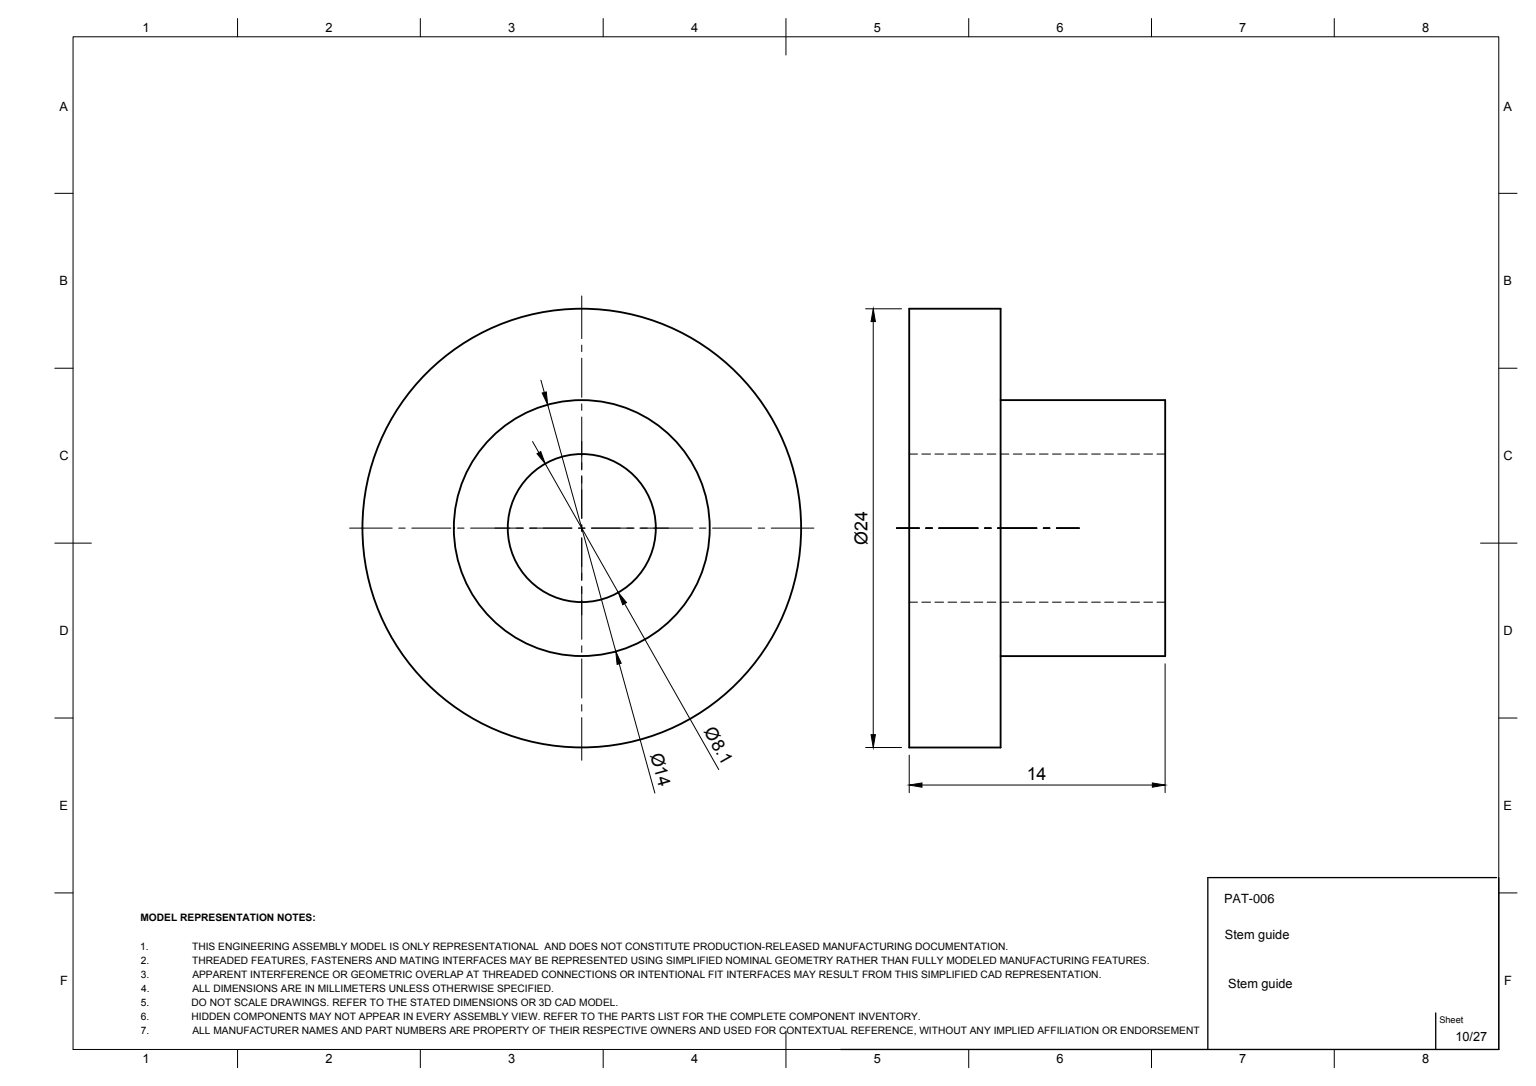
ISO-10303-21;
HEADER;
/* Generated by software containing ST-Developer
 * from STEP Tools, Inc. (www.steptools.com) 
 */

FILE_DESCRIPTION(
/* description */ ('Ball-type isolation valve (generic)'),
/* implementation_level */ '2;1');

FILE_NAME(
/* name */ 'Stem guide.step',
/* time_stamp */ '2026-10-27T10:53:05-07:00',
/* author */ (''),
/* organization */ (''),
/* preprocessor_version */ 'ST-DEVELOPER v20.2',
/* originating_system */ 'Autodesk Translation Framework v15.17.0.0',
/* authorisation */ '');

FILE_SCHEMA (('AUTOMOTIVE_DESIGN { 1 0 10303 214 3 1 1 }'));
ENDSEC;

DATA;
#10=MECHANICAL_DESIGN_GEOMETRIC_PRESENTATION_REPRESENTATION('',(#282),#7425);
#230=SHAPE_REPRESENTATION_RELATIONSHIP('SRR','None',#7540,#256);
#256=ADVANCED_BREP_SHAPE_REPRESENTATION('',(#308),#7403);
#282=STYLED_ITEM('',(#7737),#308);
#308=MANIFOLD_SOLID_BREP('Body1',#4087);
#373=FACE_BOUND('',#939,.T.);
#374=FACE_BOUND('',#942,.T.);
#375=FACE_BOUND('',#946,.T.);
#456=PLANE('',#4536);
#457=PLANE('',#4541);
#458=PLANE('',#4547);
#647=FACE_OUTER_BOUND('',#938,.T.);
#648=FACE_OUTER_BOUND('',#940,.T.);
#649=FACE_OUTER_BOUND('',#941,.T.);
#650=FACE_OUTER_BOUND('',#943,.T.);
#651=FACE_OUTER_BOUND('',#944,.T.);
#652=FACE_OUTER_BOUND('',#945,.T.);
#938=EDGE_LOOP('',(#3071));
#939=EDGE_LOOP('',(#3072));
#940=EDGE_LOOP('',(#3073,#3074,#3075,#3076));
#941=EDGE_LOOP('',(#3077));
#942=EDGE_LOOP('',(#3078));
#943=EDGE_LOOP('',(#3079,#3080,#3081,#3082));
#944=EDGE_LOOP('',(#3083,#3084,#3085,#3086));
#945=EDGE_LOOP('',(#3087));
#946=EDGE_LOOP('',(#3088));
#1251=LINE('',#6532,#1559);
#1252=LINE('',#6538,#1560);
#1253=LINE('',#6542,#1561);
#1559=VECTOR('',#5268,1.2);
#1560=VECTOR('',#5275,0.405);
#1561=VECTOR('',#5280,0.7);
#1843=CIRCLE('',#4537,1.2);
#1844=CIRCLE('',#4538,0.7);
#1845=CIRCLE('',#4540,1.2);
#1846=CIRCLE('',#4542,0.405);
#1847=CIRCLE('',#4544,0.405);
#1848=CIRCLE('',#4546,0.7);
#2056=VERTEX_POINT('',#6525);
#2057=VERTEX_POINT('',#6527);
#2058=VERTEX_POINT('',#6530);
#2059=VERTEX_POINT('',#6534);
#2060=VERTEX_POINT('',#6537);
#2061=VERTEX_POINT('',#6541);
#2428=EDGE_CURVE('',#2056,#2056,#1843,.T.);
#2429=EDGE_CURVE('',#2057,#2057,#1844,.T.);
#2430=EDGE_CURVE('',#2058,#2058,#1845,.T.);
#2431=EDGE_CURVE('',#2058,#2056,#1251,.T.);
#2432=EDGE_CURVE('',#2059,#2059,#1846,.T.);
#2433=EDGE_CURVE('',#2059,#2060,#1252,.T.);
#2434=EDGE_CURVE('',#2060,#2060,#1847,.T.);
#2435=EDGE_CURVE('',#2057,#2061,#1253,.T.);
#2436=EDGE_CURVE('',#2061,#2061,#1848,.T.);
#3071=ORIENTED_EDGE('',*,*,#2428,.F.);
#3072=ORIENTED_EDGE('',*,*,#2429,.T.);
#3073=ORIENTED_EDGE('',*,*,#2430,.F.);
#3074=ORIENTED_EDGE('',*,*,#2431,.T.);
#3075=ORIENTED_EDGE('',*,*,#2428,.T.);
#3076=ORIENTED_EDGE('',*,*,#2431,.F.);
#3077=ORIENTED_EDGE('',*,*,#2430,.T.);
#3078=ORIENTED_EDGE('',*,*,#2432,.T.);
#3079=ORIENTED_EDGE('',*,*,#2432,.F.);
#3080=ORIENTED_EDGE('',*,*,#2433,.T.);
#3081=ORIENTED_EDGE('',*,*,#2434,.T.);
#3082=ORIENTED_EDGE('',*,*,#2433,.F.);
#3083=ORIENTED_EDGE('',*,*,#2429,.F.);
#3084=ORIENTED_EDGE('',*,*,#2435,.T.);
#3085=ORIENTED_EDGE('',*,*,#2436,.T.);
#3086=ORIENTED_EDGE('',*,*,#2435,.F.);
#3087=ORIENTED_EDGE('',*,*,#2436,.F.);
#3088=ORIENTED_EDGE('',*,*,#2434,.F.);
#3792=CYLINDRICAL_SURFACE('',#4539,1.2);
#3793=CYLINDRICAL_SURFACE('',#4543,0.405);
#3794=CYLINDRICAL_SURFACE('',#4545,0.7);
#3901=ADVANCED_FACE('',(#647,#373),#456,.F.);
#3902=ADVANCED_FACE('',(#648),#3792,.T.);
#3903=ADVANCED_FACE('',(#649,#374),#457,.T.);
#3904=ADVANCED_FACE('',(#650),#3793,.F.);
#3905=ADVANCED_FACE('',(#651),#3794,.T.);
#3906=ADVANCED_FACE('',(#652,#375),#458,.F.);
#4087=CLOSED_SHELL('',(#3901,#3902,#3903,#3904,#3905,#3906));
#4535=AXIS2_PLACEMENT_3D('',#6523,#5256,#5257);
#4536=AXIS2_PLACEMENT_3D('',#6524,#5258,#5259);
#4537=AXIS2_PLACEMENT_3D('',#6526,#5260,#5261);
#4538=AXIS2_PLACEMENT_3D('',#6528,#5262,#5263);
#4539=AXIS2_PLACEMENT_3D('',#6529,#5264,#5265);
#4540=AXIS2_PLACEMENT_3D('',#6531,#5266,#5267);
#4541=AXIS2_PLACEMENT_3D('',#6533,#5269,#5270);
#4542=AXIS2_PLACEMENT_3D('',#6535,#5271,#5272);
#4543=AXIS2_PLACEMENT_3D('',#6536,#5273,#5274);
#4544=AXIS2_PLACEMENT_3D('',#6539,#5276,#5277);
#4545=AXIS2_PLACEMENT_3D('',#6540,#5278,#5279);
#4546=AXIS2_PLACEMENT_3D('',#6543,#5281,#5282);
#4547=AXIS2_PLACEMENT_3D('',#6544,#5283,#5284);
#5256=DIRECTION('axis',(0.,0.,1.));
#5257=DIRECTION('refdir',(1.,0.,0.));
#5258=DIRECTION('center_axis',(0.,0.,1.));
#5259=DIRECTION('ref_axis',(1.,0.,0.));
#5260=DIRECTION('center_axis',(0.,0.,1.));
#5261=DIRECTION('ref_axis',(1.,0.,0.));
#5262=DIRECTION('center_axis',(0.,0.,1.));
#5263=DIRECTION('ref_axis',(1.,0.,0.));
#5264=DIRECTION('center_axis',(0.,0.,1.));
#5265=DIRECTION('ref_axis',(1.,0.,0.));
#5266=DIRECTION('center_axis',(0.,0.,1.));
#5267=DIRECTION('ref_axis',(1.,0.,0.));
#5268=DIRECTION('',(0.,0.,-1.));
#5269=DIRECTION('center_axis',(0.,0.,1.));
#5270=DIRECTION('ref_axis',(1.,0.,0.));
#5271=DIRECTION('center_axis',(0.,0.,-1.));
#5272=DIRECTION('ref_axis',(1.,0.,0.));
#5273=DIRECTION('center_axis',(0.,0.,1.));
#5274=DIRECTION('ref_axis',(1.,0.,0.));
#5275=DIRECTION('',(0.,0.,-1.));
#5276=DIRECTION('center_axis',(0.,0.,-1.));
#5277=DIRECTION('ref_axis',(1.,0.,0.));
#5278=DIRECTION('center_axis',(0.,0.,1.));
#5279=DIRECTION('ref_axis',(1.,0.,0.));
#5280=DIRECTION('',(0.,0.,-1.));
#5281=DIRECTION('center_axis',(0.,0.,1.));
#5282=DIRECTION('ref_axis',(1.,0.,0.));
#5283=DIRECTION('center_axis',(0.,0.,1.));
#5284=DIRECTION('ref_axis',(1.,0.,0.));
#6523=CARTESIAN_POINT('',(0.,0.,0.));
#6524=CARTESIAN_POINT('Origin',(0.,0.,7.5));
#6525=CARTESIAN_POINT('',(-1.2,-1.46957615897682E-16,7.5));
#6526=CARTESIAN_POINT('Origin',(0.,0.,7.5));
#6527=CARTESIAN_POINT('',(-0.7,-8.57252759403147E-17,7.5));
#6528=CARTESIAN_POINT('Origin',(0.,0.,7.5));
#6529=CARTESIAN_POINT('Origin',(0.,0.,7.5));
#6530=CARTESIAN_POINT('',(-1.2,-1.46957615897682E-16,8.));
#6531=CARTESIAN_POINT('Origin',(0.,0.,8.));
#6532=CARTESIAN_POINT('',(-1.2,-1.46957615897682E-16,7.5));
#6533=CARTESIAN_POINT('Origin',(0.,0.,8.));
#6534=CARTESIAN_POINT('',(-0.405,-4.95981953654678E-17,8.));
#6535=CARTESIAN_POINT('Origin',(0.,0.,8.));
#6536=CARTESIAN_POINT('Origin',(0.,0.,6.6));
#6537=CARTESIAN_POINT('',(-0.405,-4.95981953654678E-17,6.6));
#6538=CARTESIAN_POINT('',(-0.405,-4.95981953654678E-17,6.6));
#6539=CARTESIAN_POINT('Origin',(0.,0.,6.6));
#6540=CARTESIAN_POINT('Origin',(0.,0.,6.6));
#6541=CARTESIAN_POINT('',(-0.7,-8.57252759403147E-17,6.6));
#6542=CARTESIAN_POINT('',(-0.7,-8.57252759403147E-17,6.6));
#6543=CARTESIAN_POINT('Origin',(0.,0.,6.6));
#6544=CARTESIAN_POINT('Origin',(0.,0.,6.6));
#7373=UNCERTAINTY_MEASURE_WITH_UNIT(LENGTH_MEASURE(0.001),#7426,
'DISTANCE_ACCURACY_VALUE',
'Maximum model space distance between geometric entities at asserted c
onnectivities');
#7395=UNCERTAINTY_MEASURE_WITH_UNIT(LENGTH_MEASURE(0.001),#7426,
'DISTANCE_ACCURACY_VALUE',
'Maximum model space distance between geometric entities at asserted c
onnectivities');
#7403=(
GEOMETRIC_REPRESENTATION_CONTEXT(3)
GLOBAL_UNCERTAINTY_ASSIGNED_CONTEXT((#7373))
GLOBAL_UNIT_ASSIGNED_CONTEXT((#7426,#7428,#7429))
REPRESENTATION_CONTEXT('','3D')
);
#7425=(
GEOMETRIC_REPRESENTATION_CONTEXT(3)
GLOBAL_UNCERTAINTY_ASSIGNED_CONTEXT((#7395))
GLOBAL_UNIT_ASSIGNED_CONTEXT((#7426,#7428,#7429))
REPRESENTATION_CONTEXT('','3D')
);
#7426=(
LENGTH_UNIT()
NAMED_UNIT(*)
SI_UNIT(.CENTI.,.METRE.)
);
#7428=(
NAMED_UNIT(*)
PLANE_ANGLE_UNIT()
SI_UNIT($,.RADIAN.)
);
#7429=(
NAMED_UNIT(*)
SI_UNIT($,.STERADIAN.)
SOLID_ANGLE_UNIT()
);
#7437=SHAPE_DEFINITION_REPRESENTATION(#7466,#7540);
#7466=PRODUCT_DEFINITION_SHAPE('',$,#7570);
#7540=SHAPE_REPRESENTATION('',(#4535),#7403);
#7562=PRODUCT_DEFINITION_CONTEXT('part definition',#7651,'design');
#7570=PRODUCT_DEFINITION('Stem guide','Stem guide',#7599,#7562);
#7599=PRODUCT_DEFINITION_FORMATION('',$,#7660);
#7651=APPLICATION_CONTEXT(
'Core Data for Automotive Mechanical Design Process');
#7652=PRODUCT_CONTEXT('part definition',#7651,'mechanical');
#7660=PRODUCT('Stem guide','Stem guide','Stem guide',(#7652));
#7731=COLOUR_RGB('Sky Blue',0.24,0.69,0.87);
#7732=FILL_AREA_STYLE_COLOUR('',#7731);
#7733=FILL_AREA_STYLE('',(#7732));
#7734=SURFACE_STYLE_FILL_AREA(#7733);
#7735=SURFACE_SIDE_STYLE('',(#7734));
#7736=SURFACE_STYLE_USAGE(.BOTH.,#7735);
#7737=PRESENTATION_STYLE_ASSIGNMENT((#7736));
ENDSEC;
END-ISO-10303-21;
